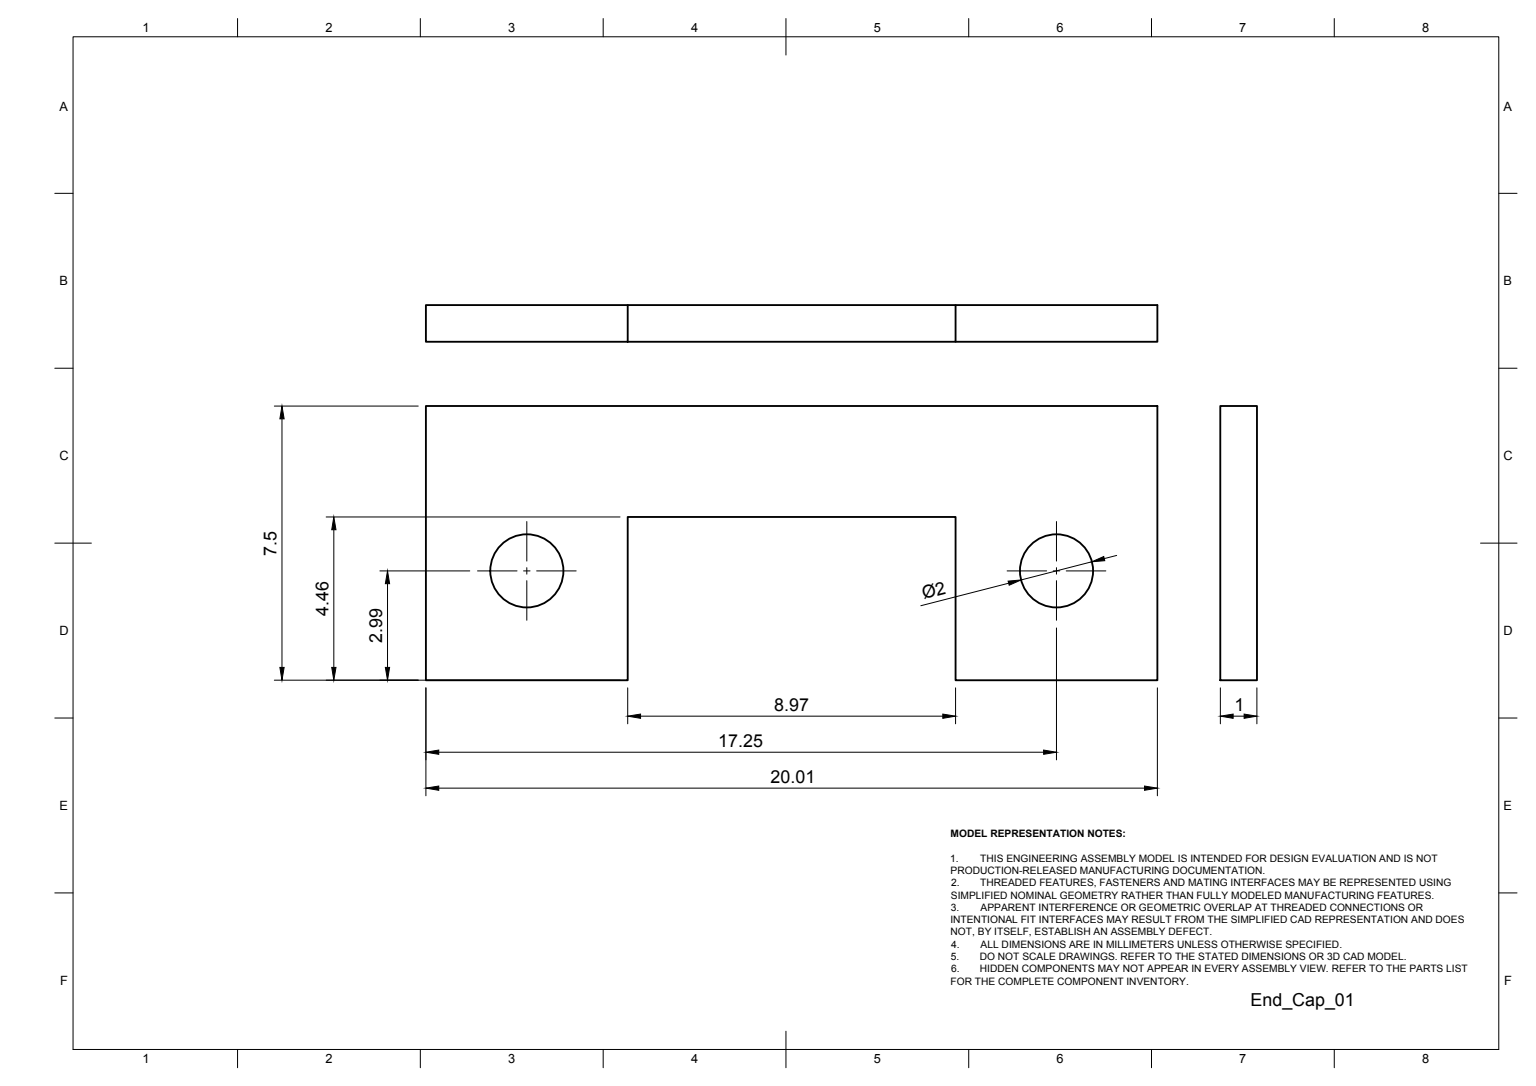
ISO-10303-21;
HEADER;
/* Generated by software containing ST-Developer
 * from STEP Tools, Inc. (www.steptools.com) 
 */

FILE_DESCRIPTION(
/* description */ (''),
/* implementation_level */ '2;1');

FILE_NAME(
/* name */ 'End_Cap_01.step',
/* time_stamp */ '2026-10-06T13:23:02-07:00',
/* author */ (''),
/* organization */ (''),
/* preprocessor_version */ 'ST-DEVELOPER v20.2',
/* originating_system */ 'Autodesk Translation Framework v15.15.0.0',
/* authorisation */ '');

FILE_SCHEMA (('AUTOMOTIVE_DESIGN { 1 0 10303 214 3 1 1 }'));
ENDSEC;

DATA;
#10=MECHANICAL_DESIGN_GEOMETRIC_PRESENTATION_REPRESENTATION('',(#78),#4994);
#58=SHAPE_REPRESENTATION_RELATIONSHIP('SRR','None',#5039,#68);
#68=ADVANCED_BREP_SHAPE_REPRESENTATION('',(#88),#4991);
#78=STYLED_ITEM('',(#5094),#88);
#88=MANIFOLD_SOLID_BREP('Body1',#2918);
#117=CYLINDRICAL_SURFACE('',#3252,1.);
#118=CYLINDRICAL_SURFACE('',#3255,1.);
#154=FACE_BOUND('',#665,.T.);
#155=FACE_BOUND('',#666,.T.);
#156=FACE_BOUND('',#668,.T.);
#157=FACE_BOUND('',#669,.T.);
#269=PLANE('',#3258);
#270=PLANE('',#3259);
#271=PLANE('',#3260);
#272=PLANE('',#3261);
#273=PLANE('',#3262);
#274=PLANE('',#3263);
#275=PLANE('',#3264);
#276=PLANE('',#3265);
#277=PLANE('',#3266);
#278=PLANE('',#3267);
#445=FACE_OUTER_BOUND('',#654,.T.);
#446=FACE_OUTER_BOUND('',#655,.T.);
#447=FACE_OUTER_BOUND('',#656,.T.);
#448=FACE_OUTER_BOUND('',#657,.T.);
#449=FACE_OUTER_BOUND('',#658,.T.);
#450=FACE_OUTER_BOUND('',#659,.T.);
#451=FACE_OUTER_BOUND('',#660,.T.);
#452=FACE_OUTER_BOUND('',#661,.T.);
#453=FACE_OUTER_BOUND('',#662,.T.);
#454=FACE_OUTER_BOUND('',#663,.T.);
#455=FACE_OUTER_BOUND('',#664,.T.);
#456=FACE_OUTER_BOUND('',#667,.T.);
#654=EDGE_LOOP('',(#2544,#2545,#2546,#2547));
#655=EDGE_LOOP('',(#2548,#2549,#2550,#2551));
#656=EDGE_LOOP('',(#2552,#2553,#2554,#2555));
#657=EDGE_LOOP('',(#2556,#2557,#2558,#2559));
#658=EDGE_LOOP('',(#2560,#2561,#2562,#2563));
#659=EDGE_LOOP('',(#2564,#2565,#2566,#2567));
#660=EDGE_LOOP('',(#2568,#2569,#2570,#2571));
#661=EDGE_LOOP('',(#2572,#2573,#2574,#2575));
#662=EDGE_LOOP('',(#2576,#2577,#2578,#2579));
#663=EDGE_LOOP('',(#2580,#2581,#2582,#2583));
#664=EDGE_LOOP('',(#2584,#2585,#2586,#2587,#2588,#2589,#2590,#2591));
#665=EDGE_LOOP('',(#2592));
#666=EDGE_LOOP('',(#2593));
#667=EDGE_LOOP('',(#2594,#2595,#2596,#2597,#2598,#2599,#2600,#2601));
#668=EDGE_LOOP('',(#2602));
#669=EDGE_LOOP('',(#2603));
#917=LINE('',#4777,#1210);
#918=LINE('',#4783,#1211);
#919=LINE('',#4788,#1212);
#920=LINE('',#4790,#1213);
#921=LINE('',#4792,#1214);
#922=LINE('',#4793,#1215);
#923=LINE('',#4796,#1216);
#924=LINE('',#4798,#1217);
#925=LINE('',#4799,#1218);
#926=LINE('',#4802,#1219);
#927=LINE('',#4804,#1220);
#928=LINE('',#4805,#1221);
#929=LINE('',#4808,#1222);
#930=LINE('',#4810,#1223);
#931=LINE('',#4811,#1224);
#932=LINE('',#4814,#1225);
#933=LINE('',#4816,#1226);
#934=LINE('',#4817,#1227);
#935=LINE('',#4820,#1228);
#936=LINE('',#4822,#1229);
#937=LINE('',#4823,#1230);
#938=LINE('',#4826,#1231);
#939=LINE('',#4828,#1232);
#940=LINE('',#4829,#1233);
#941=LINE('',#4831,#1234);
#942=LINE('',#4832,#1235);
#1210=VECTOR('',#3971,1.);
#1211=VECTOR('',#3978,1.);
#1212=VECTOR('',#3983,10.);
#1213=VECTOR('',#3984,10.);
#1214=VECTOR('',#3985,10.);
#1215=VECTOR('',#3986,10.);
#1216=VECTOR('',#3989,10.);
#1217=VECTOR('',#3990,10.);
#1218=VECTOR('',#3991,10.);
#1219=VECTOR('',#3994,10.);
#1220=VECTOR('',#3995,10.);
#1221=VECTOR('',#3996,10.);
#1222=VECTOR('',#3999,10.);
#1223=VECTOR('',#4000,10.);
#1224=VECTOR('',#4001,10.);
#1225=VECTOR('',#4004,10.);
#1226=VECTOR('',#4005,10.);
#1227=VECTOR('',#4006,10.);
#1228=VECTOR('',#4009,10.);
#1229=VECTOR('',#4010,10.);
#1230=VECTOR('',#4011,10.);
#1231=VECTOR('',#4014,10.);
#1232=VECTOR('',#4015,10.);
#1233=VECTOR('',#4016,10.);
#1234=VECTOR('',#4019,10.);
#1235=VECTOR('',#4020,10.);
#1357=CIRCLE('',#3253,1.);
#1358=CIRCLE('',#3254,1.);
#1359=CIRCLE('',#3256,1.);
#1360=CIRCLE('',#3257,1.);
#1542=VERTEX_POINT('',#4774);
#1543=VERTEX_POINT('',#4776);
#1544=VERTEX_POINT('',#4780);
#1545=VERTEX_POINT('',#4782);
#1546=VERTEX_POINT('',#4786);
#1547=VERTEX_POINT('',#4787);
#1548=VERTEX_POINT('',#4789);
#1549=VERTEX_POINT('',#4791);
#1550=VERTEX_POINT('',#4795);
#1551=VERTEX_POINT('',#4797);
#1552=VERTEX_POINT('',#4801);
#1553=VERTEX_POINT('',#4803);
#1554=VERTEX_POINT('',#4807);
#1555=VERTEX_POINT('',#4809);
#1556=VERTEX_POINT('',#4813);
#1557=VERTEX_POINT('',#4815);
#1558=VERTEX_POINT('',#4819);
#1559=VERTEX_POINT('',#4821);
#1560=VERTEX_POINT('',#4825);
#1561=VERTEX_POINT('',#4827);
#1886=EDGE_CURVE('',#1542,#1542,#1357,.T.);
#1887=EDGE_CURVE('',#1542,#1543,#917,.T.);
#1888=EDGE_CURVE('',#1543,#1543,#1358,.T.);
#1889=EDGE_CURVE('',#1544,#1544,#1359,.T.);
#1890=EDGE_CURVE('',#1544,#1545,#918,.T.);
#1891=EDGE_CURVE('',#1545,#1545,#1360,.T.);
#1892=EDGE_CURVE('',#1546,#1547,#919,.T.);
#1893=EDGE_CURVE('',#1547,#1548,#920,.T.);
#1894=EDGE_CURVE('',#1549,#1548,#921,.T.);
#1895=EDGE_CURVE('',#1546,#1549,#922,.T.);
#1896=EDGE_CURVE('',#1550,#1546,#923,.T.);
#1897=EDGE_CURVE('',#1551,#1549,#924,.T.);
#1898=EDGE_CURVE('',#1550,#1551,#925,.T.);
#1899=EDGE_CURVE('',#1552,#1550,#926,.T.);
#1900=EDGE_CURVE('',#1553,#1551,#927,.T.);
#1901=EDGE_CURVE('',#1552,#1553,#928,.T.);
#1902=EDGE_CURVE('',#1554,#1552,#929,.T.);
#1903=EDGE_CURVE('',#1555,#1553,#930,.T.);
#1904=EDGE_CURVE('',#1554,#1555,#931,.T.);
#1905=EDGE_CURVE('',#1556,#1554,#932,.T.);
#1906=EDGE_CURVE('',#1557,#1555,#933,.T.);
#1907=EDGE_CURVE('',#1556,#1557,#934,.T.);
#1908=EDGE_CURVE('',#1558,#1556,#935,.T.);
#1909=EDGE_CURVE('',#1559,#1557,#936,.T.);
#1910=EDGE_CURVE('',#1558,#1559,#937,.T.);
#1911=EDGE_CURVE('',#1560,#1558,#938,.T.);
#1912=EDGE_CURVE('',#1561,#1559,#939,.T.);
#1913=EDGE_CURVE('',#1560,#1561,#940,.T.);
#1914=EDGE_CURVE('',#1547,#1560,#941,.T.);
#1915=EDGE_CURVE('',#1548,#1561,#942,.T.);
#2544=ORIENTED_EDGE('',*,*,#1886,.F.);
#2545=ORIENTED_EDGE('',*,*,#1887,.T.);
#2546=ORIENTED_EDGE('',*,*,#1888,.F.);
#2547=ORIENTED_EDGE('',*,*,#1887,.F.);
#2548=ORIENTED_EDGE('',*,*,#1889,.F.);
#2549=ORIENTED_EDGE('',*,*,#1890,.T.);
#2550=ORIENTED_EDGE('',*,*,#1891,.F.);
#2551=ORIENTED_EDGE('',*,*,#1890,.F.);
#2552=ORIENTED_EDGE('',*,*,#1892,.T.);
#2553=ORIENTED_EDGE('',*,*,#1893,.T.);
#2554=ORIENTED_EDGE('',*,*,#1894,.F.);
#2555=ORIENTED_EDGE('',*,*,#1895,.F.);
#2556=ORIENTED_EDGE('',*,*,#1896,.T.);
#2557=ORIENTED_EDGE('',*,*,#1895,.T.);
#2558=ORIENTED_EDGE('',*,*,#1897,.F.);
#2559=ORIENTED_EDGE('',*,*,#1898,.F.);
#2560=ORIENTED_EDGE('',*,*,#1899,.T.);
#2561=ORIENTED_EDGE('',*,*,#1898,.T.);
#2562=ORIENTED_EDGE('',*,*,#1900,.F.);
#2563=ORIENTED_EDGE('',*,*,#1901,.F.);
#2564=ORIENTED_EDGE('',*,*,#1902,.T.);
#2565=ORIENTED_EDGE('',*,*,#1901,.T.);
#2566=ORIENTED_EDGE('',*,*,#1903,.F.);
#2567=ORIENTED_EDGE('',*,*,#1904,.F.);
#2568=ORIENTED_EDGE('',*,*,#1905,.T.);
#2569=ORIENTED_EDGE('',*,*,#1904,.T.);
#2570=ORIENTED_EDGE('',*,*,#1906,.F.);
#2571=ORIENTED_EDGE('',*,*,#1907,.F.);
#2572=ORIENTED_EDGE('',*,*,#1908,.T.);
#2573=ORIENTED_EDGE('',*,*,#1907,.T.);
#2574=ORIENTED_EDGE('',*,*,#1909,.F.);
#2575=ORIENTED_EDGE('',*,*,#1910,.F.);
#2576=ORIENTED_EDGE('',*,*,#1911,.T.);
#2577=ORIENTED_EDGE('',*,*,#1910,.T.);
#2578=ORIENTED_EDGE('',*,*,#1912,.F.);
#2579=ORIENTED_EDGE('',*,*,#1913,.F.);
#2580=ORIENTED_EDGE('',*,*,#1914,.T.);
#2581=ORIENTED_EDGE('',*,*,#1913,.T.);
#2582=ORIENTED_EDGE('',*,*,#1915,.F.);
#2583=ORIENTED_EDGE('',*,*,#1893,.F.);
#2584=ORIENTED_EDGE('',*,*,#1915,.T.);
#2585=ORIENTED_EDGE('',*,*,#1912,.T.);
#2586=ORIENTED_EDGE('',*,*,#1909,.T.);
#2587=ORIENTED_EDGE('',*,*,#1906,.T.);
#2588=ORIENTED_EDGE('',*,*,#1903,.T.);
#2589=ORIENTED_EDGE('',*,*,#1900,.T.);
#2590=ORIENTED_EDGE('',*,*,#1897,.T.);
#2591=ORIENTED_EDGE('',*,*,#1894,.T.);
#2592=ORIENTED_EDGE('',*,*,#1886,.T.);
#2593=ORIENTED_EDGE('',*,*,#1889,.T.);
#2594=ORIENTED_EDGE('',*,*,#1914,.F.);
#2595=ORIENTED_EDGE('',*,*,#1892,.F.);
#2596=ORIENTED_EDGE('',*,*,#1896,.F.);
#2597=ORIENTED_EDGE('',*,*,#1899,.F.);
#2598=ORIENTED_EDGE('',*,*,#1902,.F.);
#2599=ORIENTED_EDGE('',*,*,#1905,.F.);
#2600=ORIENTED_EDGE('',*,*,#1908,.F.);
#2601=ORIENTED_EDGE('',*,*,#1911,.F.);
#2602=ORIENTED_EDGE('',*,*,#1888,.T.);
#2603=ORIENTED_EDGE('',*,*,#1891,.T.);
#2875=ADVANCED_FACE('',(#445),#117,.F.);
#2876=ADVANCED_FACE('',(#446),#118,.F.);
#2877=ADVANCED_FACE('',(#447),#269,.T.);
#2878=ADVANCED_FACE('',(#448),#270,.T.);
#2879=ADVANCED_FACE('',(#449),#271,.T.);
#2880=ADVANCED_FACE('',(#450),#272,.T.);
#2881=ADVANCED_FACE('',(#451),#273,.T.);
#2882=ADVANCED_FACE('',(#452),#274,.T.);
#2883=ADVANCED_FACE('',(#453),#275,.T.);
#2884=ADVANCED_FACE('',(#454),#276,.T.);
#2885=ADVANCED_FACE('',(#455,#154,#155),#277,.T.);
#2886=ADVANCED_FACE('',(#456,#156,#157),#278,.F.);
#2918=CLOSED_SHELL('',(#2875,#2876,#2877,#2878,#2879,#2880,#2881,#2882,
#2883,#2884,#2885,#2886));
#3251=AXIS2_PLACEMENT_3D('',#4772,#3965,#3966);
#3252=AXIS2_PLACEMENT_3D('',#4773,#3967,#3968);
#3253=AXIS2_PLACEMENT_3D('',#4775,#3969,#3970);
#3254=AXIS2_PLACEMENT_3D('',#4778,#3972,#3973);
#3255=AXIS2_PLACEMENT_3D('',#4779,#3974,#3975);
#3256=AXIS2_PLACEMENT_3D('',#4781,#3976,#3977);
#3257=AXIS2_PLACEMENT_3D('',#4784,#3979,#3980);
#3258=AXIS2_PLACEMENT_3D('',#4785,#3981,#3982);
#3259=AXIS2_PLACEMENT_3D('',#4794,#3987,#3988);
#3260=AXIS2_PLACEMENT_3D('',#4800,#3992,#3993);
#3261=AXIS2_PLACEMENT_3D('',#4806,#3997,#3998);
#3262=AXIS2_PLACEMENT_3D('',#4812,#4002,#4003);
#3263=AXIS2_PLACEMENT_3D('',#4818,#4007,#4008);
#3264=AXIS2_PLACEMENT_3D('',#4824,#4012,#4013);
#3265=AXIS2_PLACEMENT_3D('',#4830,#4017,#4018);
#3266=AXIS2_PLACEMENT_3D('',#4833,#4021,#4022);
#3267=AXIS2_PLACEMENT_3D('',#4834,#4023,#4024);
#3965=DIRECTION('axis',(0.,0.,1.));
#3966=DIRECTION('refdir',(1.,0.,0.));
#3967=DIRECTION('center_axis',(-1.,0.,0.));
#3968=DIRECTION('ref_axis',(0.,1.,0.));
#3969=DIRECTION('center_axis',(-1.,0.,0.));
#3970=DIRECTION('ref_axis',(0.,1.,0.));
#3971=DIRECTION('',(-1.,0.,0.));
#3972=DIRECTION('center_axis',(1.,0.,0.));
#3973=DIRECTION('ref_axis',(0.,1.,0.));
#3974=DIRECTION('center_axis',(-1.,0.,0.));
#3975=DIRECTION('ref_axis',(0.,1.,0.));
#3976=DIRECTION('center_axis',(-1.,0.,0.));
#3977=DIRECTION('ref_axis',(0.,1.,0.));
#3978=DIRECTION('',(-1.,0.,0.));
#3979=DIRECTION('center_axis',(1.,0.,0.));
#3980=DIRECTION('ref_axis',(0.,1.,0.));
#3981=DIRECTION('center_axis',(0.,1.,0.));
#3982=DIRECTION('ref_axis',(0.,0.,1.));
#3983=DIRECTION('',(0.,0.,1.));
#3984=DIRECTION('',(1.,0.,0.));
#3985=DIRECTION('',(0.,0.,1.));
#3986=DIRECTION('',(1.,0.,0.));
#3987=DIRECTION('center_axis',(0.,0.,-1.));
#3988=DIRECTION('ref_axis',(0.,1.,0.));
#3989=DIRECTION('',(0.,1.,0.));
#3990=DIRECTION('',(0.,1.,0.));
#3991=DIRECTION('',(1.,0.,0.));
#3992=DIRECTION('center_axis',(0.,-1.,0.));
#3993=DIRECTION('ref_axis',(0.,0.,-1.));
#3994=DIRECTION('',(0.,0.,-1.));
#3995=DIRECTION('',(0.,0.,-1.));
#3996=DIRECTION('',(1.,0.,0.));
#3997=DIRECTION('center_axis',(0.,0.,-1.));
#3998=DIRECTION('ref_axis',(0.,1.,0.));
#3999=DIRECTION('',(0.,1.,0.));
#4000=DIRECTION('',(0.,1.,0.));
#4001=DIRECTION('',(1.,0.,0.));
#4002=DIRECTION('center_axis',(0.,1.,0.));
#4003=DIRECTION('ref_axis',(0.,0.,1.));
#4004=DIRECTION('',(0.,0.,1.));
#4005=DIRECTION('',(0.,0.,1.));
#4006=DIRECTION('',(1.,0.,0.));
#4007=DIRECTION('center_axis',(0.,0.,-1.));
#4008=DIRECTION('ref_axis',(0.,1.,0.));
#4009=DIRECTION('',(0.,1.,0.));
#4010=DIRECTION('',(0.,1.,0.));
#4011=DIRECTION('',(1.,0.,0.));
#4012=DIRECTION('center_axis',(0.,-1.,0.));
#4013=DIRECTION('ref_axis',(0.,0.,-1.));
#4014=DIRECTION('',(0.,0.,-1.));
#4015=DIRECTION('',(0.,0.,-1.));
#4016=DIRECTION('',(1.,0.,0.));
#4017=DIRECTION('center_axis',(0.,0.,1.));
#4018=DIRECTION('ref_axis',(0.,-1.,0.));
#4019=DIRECTION('',(0.,-1.,0.));
#4020=DIRECTION('',(0.,-1.,0.));
#4021=DIRECTION('center_axis',(1.,0.,0.));
#4022=DIRECTION('ref_axis',(0.,0.,-1.));
#4023=DIRECTION('center_axis',(1.,0.,0.));
#4024=DIRECTION('ref_axis',(0.,1.,0.));
#4772=CARTESIAN_POINT('',(0.,0.,0.));
#4773=CARTESIAN_POINT('Origin',(14.5,7.24395366693103,1.75498192028357));
#4774=CARTESIAN_POINT('',(14.5,6.24395366693103,1.75498192028357));
#4775=CARTESIAN_POINT('Origin',(14.5,7.24395366693103,1.75498192028357));
#4776=CARTESIAN_POINT('',(13.5,6.24395366693103,1.75498192028357));
#4777=CARTESIAN_POINT('',(14.5,6.24395366693103,1.75498192028357));
#4778=CARTESIAN_POINT('Origin',(13.5,7.24395366693103,1.75498192028357));
#4779=CARTESIAN_POINT('Origin',(14.5,-7.24395366693103,1.75498192028357));
#4780=CARTESIAN_POINT('',(14.5,-8.24395366693103,1.75498192028357));
#4781=CARTESIAN_POINT('Origin',(14.5,-7.24395366693103,1.75498192028357));
#4782=CARTESIAN_POINT('',(13.5,-8.24395366693103,1.75498192028357));
#4783=CARTESIAN_POINT('',(14.5,-8.24395366693103,1.75498192028357));
#4784=CARTESIAN_POINT('Origin',(13.5,-7.24395366693103,1.75498192028357));
#4785=CARTESIAN_POINT('Origin',(13.5,10.0039433906299,-1.2346845122375));
#4786=CARTESIAN_POINT('',(13.5,10.0039433906299,-1.2346845122375));
#4787=CARTESIAN_POINT('',(13.5,10.0039433906299,6.26348125396711));
#4788=CARTESIAN_POINT('',(13.5,10.0039433906299,-1.2346845122375));
#4789=CARTESIAN_POINT('',(14.5,10.0039433906299,6.26348125396711));
#4790=CARTESIAN_POINT('',(13.5,10.0039433906299,6.26348125396711));
#4791=CARTESIAN_POINT('',(14.5,10.0039433906299,-1.2346845122375));
#4792=CARTESIAN_POINT('',(14.5,10.0039433906299,-1.2346845122375));
#4793=CARTESIAN_POINT('',(13.5,10.0039433906299,-1.2346845122375));
#4794=CARTESIAN_POINT('Origin',(13.5,4.48396394323217,-1.2346845122375));
#4795=CARTESIAN_POINT('',(13.5,4.48396394323217,-1.2346845122375));
#4796=CARTESIAN_POINT('',(13.5,4.48396394323217,-1.2346845122375));
#4797=CARTESIAN_POINT('',(14.5,4.48396394323217,-1.2346845122375));
#4798=CARTESIAN_POINT('',(14.5,4.48396394323217,-1.2346845122375));
#4799=CARTESIAN_POINT('',(13.5,4.48396394323217,-1.2346845122375));
#4800=CARTESIAN_POINT('Origin',(13.5,4.48396394323217,3.23022961141938));
#4801=CARTESIAN_POINT('',(13.5,4.48396394323217,3.23022961141938));
#4802=CARTESIAN_POINT('',(13.5,4.48396394323217,3.23022961141938));
#4803=CARTESIAN_POINT('',(14.5,4.48396394323217,3.23022961141938));
#4804=CARTESIAN_POINT('',(14.5,4.48396394323217,3.23022961141938));
#4805=CARTESIAN_POINT('',(13.5,4.48396394323217,3.23022961141938));
#4806=CARTESIAN_POINT('Origin',(13.5,-4.48396394323217,3.23022961141938));
#4807=CARTESIAN_POINT('',(13.5,-4.48396394323217,3.23022961141938));
#4808=CARTESIAN_POINT('',(13.5,-4.48396394323217,3.23022961141938));
#4809=CARTESIAN_POINT('',(14.5,-4.48396394323217,3.23022961141938));
#4810=CARTESIAN_POINT('',(14.5,-4.48396394323217,3.23022961141938));
#4811=CARTESIAN_POINT('',(13.5,-4.48396394323217,3.23022961141938));
#4812=CARTESIAN_POINT('Origin',(13.5,-4.48396394323217,-1.2346845122375));
#4813=CARTESIAN_POINT('',(13.5,-4.48396394323217,-1.2346845122375));
#4814=CARTESIAN_POINT('',(13.5,-4.48396394323217,-1.2346845122375));
#4815=CARTESIAN_POINT('',(14.5,-4.48396394323217,-1.2346845122375));
#4816=CARTESIAN_POINT('',(14.5,-4.48396394323217,-1.2346845122375));
#4817=CARTESIAN_POINT('',(13.5,-4.48396394323217,-1.2346845122375));
#4818=CARTESIAN_POINT('Origin',(13.5,-10.0039433906299,-1.2346845122375));
#4819=CARTESIAN_POINT('',(13.5,-10.0039433906299,-1.2346845122375));
#4820=CARTESIAN_POINT('',(13.5,-10.0039433906299,-1.2346845122375));
#4821=CARTESIAN_POINT('',(14.5,-10.0039433906299,-1.2346845122375));
#4822=CARTESIAN_POINT('',(14.5,-10.0039433906299,-1.2346845122375));
#4823=CARTESIAN_POINT('',(13.5,-10.0039433906299,-1.2346845122375));
#4824=CARTESIAN_POINT('Origin',(13.5,-10.0039433906299,6.26348125396711));
#4825=CARTESIAN_POINT('',(13.5,-10.0039433906299,6.26348125396711));
#4826=CARTESIAN_POINT('',(13.5,-10.0039433906299,6.26348125396711));
#4827=CARTESIAN_POINT('',(14.5,-10.0039433906299,6.26348125396711));
#4828=CARTESIAN_POINT('',(14.5,-10.0039433906299,6.26348125396711));
#4829=CARTESIAN_POINT('',(13.5,-10.0039433906299,6.26348125396711));
#4830=CARTESIAN_POINT('Origin',(13.5,10.0039433906299,6.26348125396711));
#4831=CARTESIAN_POINT('',(13.5,10.0039433906299,6.26348125396711));
#4832=CARTESIAN_POINT('',(14.5,10.0039433906299,6.26348125396711));
#4833=CARTESIAN_POINT('Origin',(14.5,0.,2.51439837086481));
#4834=CARTESIAN_POINT('Origin',(13.5,0.,2.51439837086481));
#4979=UNCERTAINTY_MEASURE_WITH_UNIT(LENGTH_MEASURE(0.01),#4995,
'DISTANCE_ACCURACY_VALUE',
'Maximum model space distance between geometric entities at asserted c
onnectivities');
#4982=UNCERTAINTY_MEASURE_WITH_UNIT(LENGTH_MEASURE(0.01),#4995,
'DISTANCE_ACCURACY_VALUE',
'Maximum model space distance between geometric entities at asserted c
onnectivities');
#4991=(
GEOMETRIC_REPRESENTATION_CONTEXT(3)
GLOBAL_UNCERTAINTY_ASSIGNED_CONTEXT((#4979))
GLOBAL_UNIT_ASSIGNED_CONTEXT((#4995,#4997,#4998))
REPRESENTATION_CONTEXT('','3D')
);
#4994=(
GEOMETRIC_REPRESENTATION_CONTEXT(3)
GLOBAL_UNCERTAINTY_ASSIGNED_CONTEXT((#4982))
GLOBAL_UNIT_ASSIGNED_CONTEXT((#4995,#4997,#4998))
REPRESENTATION_CONTEXT('','3D')
);
#4995=(
LENGTH_UNIT()
NAMED_UNIT(*)
SI_UNIT(.MILLI.,.METRE.)
);
#4997=(
NAMED_UNIT(*)
PLANE_ANGLE_UNIT()
SI_UNIT($,.RADIAN.)
);
#4998=(
NAMED_UNIT(*)
SI_UNIT($,.STERADIAN.)
SOLID_ANGLE_UNIT()
);
#5007=SHAPE_DEFINITION_REPRESENTATION(#5018,#5039);
#5018=PRODUCT_DEFINITION_SHAPE('',$,#5051);
#5039=SHAPE_REPRESENTATION('',(#3251),#4991);
#5042=PRODUCT_DEFINITION_CONTEXT('part definition',#5077,'design');
#5051=PRODUCT_DEFINITION('End_Cap_01','End_Cap_01',#5062,#5042);
#5062=PRODUCT_DEFINITION_FORMATION('',$,#5087);
#5077=APPLICATION_CONTEXT(
'Core Data for Automotive Mechanical Design Process');
#5078=PRODUCT_CONTEXT('part definition',#5077,'mechanical');
#5087=PRODUCT('End_Cap_01','End_Cap_01',$,(#5078));
#5094=PRESENTATION_STYLE_ASSIGNMENT((#5099));
#5099=SURFACE_STYLE_USAGE(.BOTH.,#5104);
#5104=SURFACE_SIDE_STYLE('',(#5109));
#5109=SURFACE_STYLE_FILL_AREA(#5114);
#5114=FILL_AREA_STYLE('Opaque(196,0,0)',(#5119));
#5119=FILL_AREA_STYLE_COLOUR('Opaque(196,0,0)',#5124);
#5124=COLOUR_RGB('Opaque(196,0,0)', 0.66274510, 0.83137255, 0.94901961);
ENDSEC;
END-ISO-10303-21;
